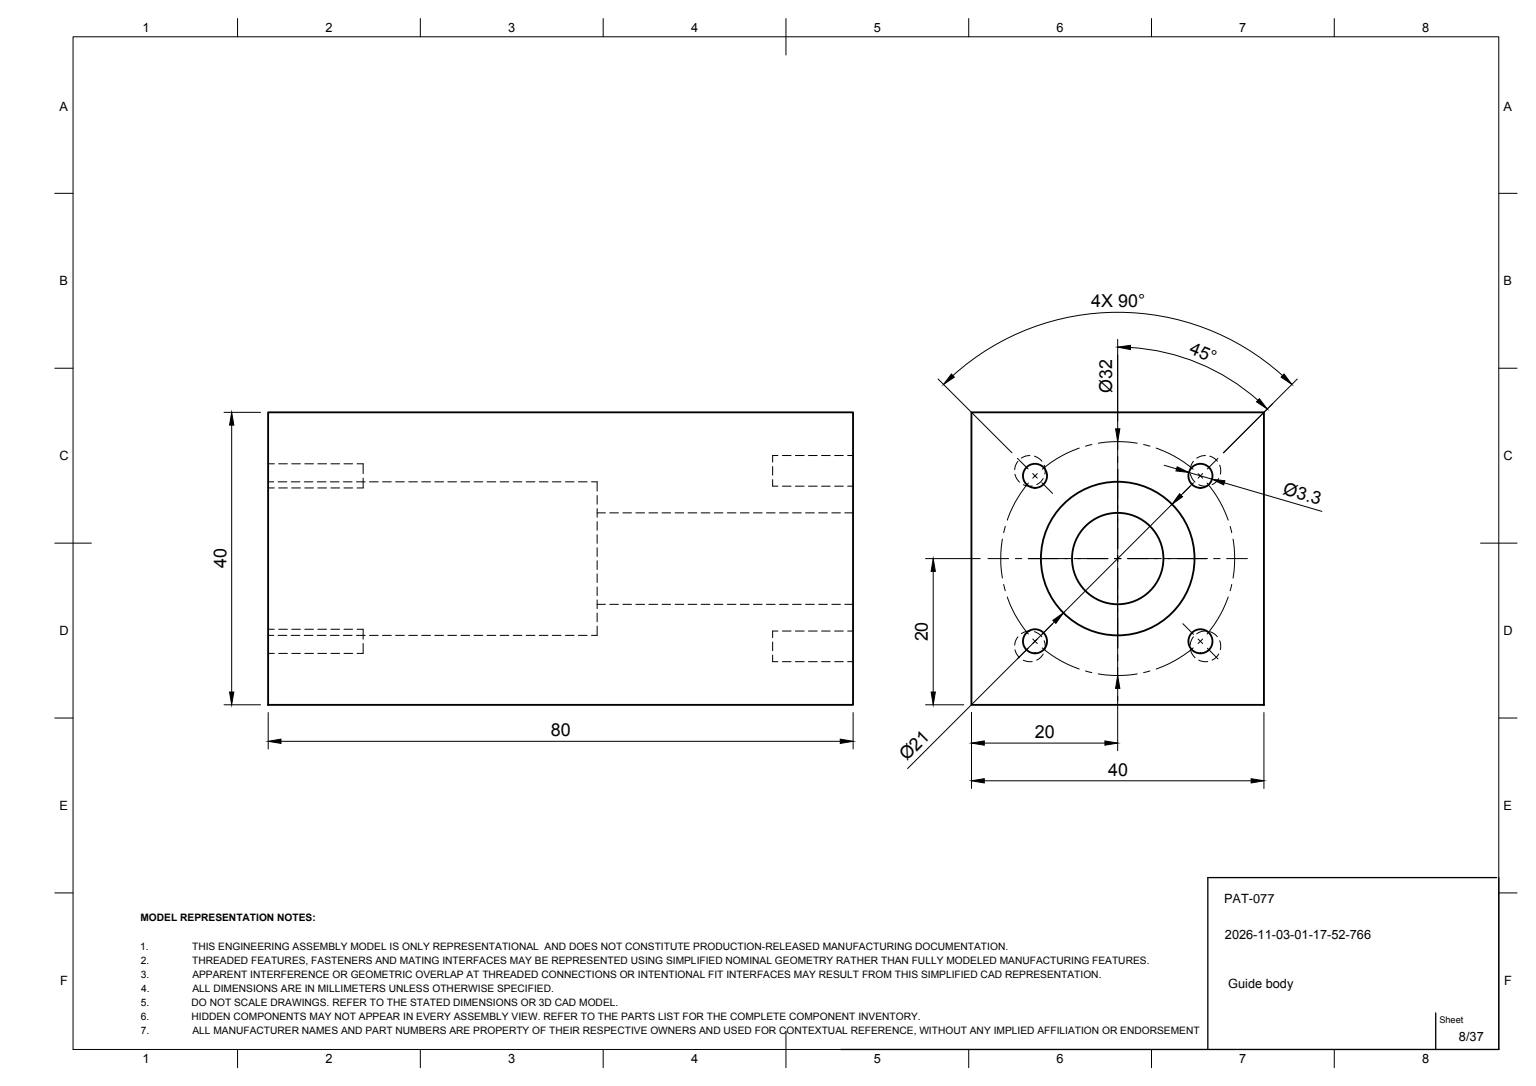
ISO-10303-21;
HEADER;
/* Generated by software containing ST-Developer
 * from STEP Tools, Inc. (www.steptools.com) 
 */

FILE_DESCRIPTION(
/* description */ ('Pallet stop with pneumatic fitting'),
/* implementation_level */ '2;1');

FILE_NAME(
/* name */ 'Guide body.step',
/* time_stamp */ '2026-10-27T10:51:41-07:00',
/* author */ (''),
/* organization */ (''),
/* preprocessor_version */ 'ST-DEVELOPER v20.2',
/* originating_system */ 'Autodesk Translation Framework v15.17.0.0',
/* authorisation */ '');

FILE_SCHEMA (('AUTOMOTIVE_DESIGN { 1 0 10303 214 3 1 1 }'));
ENDSEC;

DATA;
#10=MECHANICAL_DESIGN_GEOMETRIC_PRESENTATION_REPRESENTATION('',(#360),#10265);
#296=SHAPE_REPRESENTATION_RELATIONSHIP('SRR','None',#10409,#328);
#328=ADVANCED_BREP_SHAPE_REPRESENTATION('',(#392),#10233);
#360=STYLED_ITEM('',(#10634),#392);
#392=MANIFOLD_SOLID_BREP('Body1',#5048);
#437=FACE_BOUND('',#1113,.T.);
#438=FACE_BOUND('',#1120,.T.);
#439=FACE_BOUND('',#1121,.T.);
#440=FACE_BOUND('',#1122,.T.);
#441=FACE_BOUND('',#1123,.T.);
#442=FACE_BOUND('',#1124,.T.);
#443=FACE_BOUND('',#1126,.T.);
#444=FACE_BOUND('',#1127,.T.);
#445=FACE_BOUND('',#1128,.T.);
#446=FACE_BOUND('',#1129,.T.);
#447=FACE_BOUND('',#1130,.T.);
#563=PLANE('',#5486);
#564=PLANE('',#5490);
#565=PLANE('',#5494);
#566=PLANE('',#5498);
#567=PLANE('',#5502);
#568=PLANE('',#5506);
#569=PLANE('',#5510);
#570=PLANE('',#5514);
#571=PLANE('',#5518);
#572=PLANE('',#5522);
#573=PLANE('',#5523);
#574=PLANE('',#5524);
#575=PLANE('',#5525);
#576=PLANE('',#5526);
#577=PLANE('',#5527);
#763=FACE_OUTER_BOUND('',#1095,.T.);
#764=FACE_OUTER_BOUND('',#1096,.T.);
#765=FACE_OUTER_BOUND('',#1097,.T.);
#766=FACE_OUTER_BOUND('',#1098,.T.);
#767=FACE_OUTER_BOUND('',#1099,.T.);
#768=FACE_OUTER_BOUND('',#1100,.T.);
#769=FACE_OUTER_BOUND('',#1101,.T.);
#770=FACE_OUTER_BOUND('',#1102,.T.);
#771=FACE_OUTER_BOUND('',#1103,.T.);
#772=FACE_OUTER_BOUND('',#1104,.T.);
#773=FACE_OUTER_BOUND('',#1105,.T.);
#774=FACE_OUTER_BOUND('',#1106,.T.);
#775=FACE_OUTER_BOUND('',#1107,.T.);
#776=FACE_OUTER_BOUND('',#1108,.T.);
#777=FACE_OUTER_BOUND('',#1109,.T.);
#778=FACE_OUTER_BOUND('',#1110,.T.);
#779=FACE_OUTER_BOUND('',#1111,.T.);
#780=FACE_OUTER_BOUND('',#1112,.T.);
#781=FACE_OUTER_BOUND('',#1114,.T.);
#782=FACE_OUTER_BOUND('',#1115,.T.);
#783=FACE_OUTER_BOUND('',#1116,.T.);
#784=FACE_OUTER_BOUND('',#1117,.T.);
#785=FACE_OUTER_BOUND('',#1118,.T.);
#786=FACE_OUTER_BOUND('',#1119,.T.);
#787=FACE_OUTER_BOUND('',#1125,.T.);
#1095=EDGE_LOOP('',(#3536,#3537,#3538,#3539));
#1096=EDGE_LOOP('',(#3540));
#1097=EDGE_LOOP('',(#3541,#3542,#3543,#3544));
#1098=EDGE_LOOP('',(#3545));
#1099=EDGE_LOOP('',(#3546,#3547,#3548,#3549));
#1100=EDGE_LOOP('',(#3550));
#1101=EDGE_LOOP('',(#3551,#3552,#3553,#3554));
#1102=EDGE_LOOP('',(#3555));
#1103=EDGE_LOOP('',(#3556,#3557,#3558,#3559));
#1104=EDGE_LOOP('',(#3560));
#1105=EDGE_LOOP('',(#3561,#3562,#3563,#3564));
#1106=EDGE_LOOP('',(#3565));
#1107=EDGE_LOOP('',(#3566,#3567,#3568,#3569));
#1108=EDGE_LOOP('',(#3570));
#1109=EDGE_LOOP('',(#3571,#3572,#3573,#3574));
#1110=EDGE_LOOP('',(#3575));
#1111=EDGE_LOOP('',(#3576,#3577,#3578,#3579));
#1112=EDGE_LOOP('',(#3580));
#1113=EDGE_LOOP('',(#3581));
#1114=EDGE_LOOP('',(#3582,#3583,#3584,#3585));
#1115=EDGE_LOOP('',(#3586,#3587,#3588,#3589));
#1116=EDGE_LOOP('',(#3590,#3591,#3592,#3593));
#1117=EDGE_LOOP('',(#3594,#3595,#3596,#3597));
#1118=EDGE_LOOP('',(#3598,#3599,#3600,#3601));
#1119=EDGE_LOOP('',(#3602,#3603,#3604,#3605));
#1120=EDGE_LOOP('',(#3606));
#1121=EDGE_LOOP('',(#3607));
#1122=EDGE_LOOP('',(#3608));
#1123=EDGE_LOOP('',(#3609));
#1124=EDGE_LOOP('',(#3610));
#1125=EDGE_LOOP('',(#3611,#3612,#3613,#3614));
#1126=EDGE_LOOP('',(#3615));
#1127=EDGE_LOOP('',(#3616));
#1128=EDGE_LOOP('',(#3617));
#1129=EDGE_LOOP('',(#3618));
#1130=EDGE_LOOP('',(#3619));
#1535=LINE('',#7880,#1870);
#1536=LINE('',#7887,#1871);
#1537=LINE('',#7894,#1872);
#1538=LINE('',#7901,#1873);
#1539=LINE('',#7908,#1874);
#1540=LINE('',#7915,#1875);
#1541=LINE('',#7922,#1876);
#1542=LINE('',#7929,#1877);
#1543=LINE('',#7936,#1878);
#1544=LINE('',#7944,#1879);
#1545=LINE('',#7948,#1880);
#1546=LINE('',#7950,#1881);
#1547=LINE('',#7952,#1882);
#1548=LINE('',#7953,#1883);
#1549=LINE('',#7956,#1884);
#1550=LINE('',#7958,#1885);
#1551=LINE('',#7959,#1886);
#1552=LINE('',#7962,#1887);
#1553=LINE('',#7964,#1888);
#1554=LINE('',#7965,#1889);
#1555=LINE('',#7967,#1890);
#1556=LINE('',#7968,#1891);
#1870=VECTOR('',#6240,0.165);
#1871=VECTOR('',#6249,0.165);
#1872=VECTOR('',#6258,0.165);
#1873=VECTOR('',#6267,0.165);
#1874=VECTOR('',#6276,0.21);
#1875=VECTOR('',#6285,0.21);
#1876=VECTOR('',#6294,0.21);
#1877=VECTOR('',#6303,0.21);
#1878=VECTOR('',#6312,1.05);
#1879=VECTOR('',#6323,0.625);
#1880=VECTOR('',#6326,1.);
#1881=VECTOR('',#6327,1.);
#1882=VECTOR('',#6328,1.);
#1883=VECTOR('',#6329,1.);
#1884=VECTOR('',#6332,1.);
#1885=VECTOR('',#6333,1.);
#1886=VECTOR('',#6334,1.);
#1887=VECTOR('',#6337,1.);
#1888=VECTOR('',#6338,1.);
#1889=VECTOR('',#6339,1.);
#1890=VECTOR('',#6342,1.);
#1891=VECTOR('',#6343,1.);
#2178=CIRCLE('',#5484,0.165);
#2179=CIRCLE('',#5485,0.165);
#2180=CIRCLE('',#5488,0.165);
#2181=CIRCLE('',#5489,0.165);
#2182=CIRCLE('',#5492,0.165);
#2183=CIRCLE('',#5493,0.165);
#2184=CIRCLE('',#5496,0.165);
#2185=CIRCLE('',#5497,0.165);
#2186=CIRCLE('',#5500,0.21);
#2187=CIRCLE('',#5501,0.21);
#2188=CIRCLE('',#5504,0.21);
#2189=CIRCLE('',#5505,0.21);
#2190=CIRCLE('',#5508,0.21);
#2191=CIRCLE('',#5509,0.21);
#2192=CIRCLE('',#5512,0.21);
#2193=CIRCLE('',#5513,0.21);
#2194=CIRCLE('',#5516,1.05);
#2195=CIRCLE('',#5517,1.05);
#2196=CIRCLE('',#5519,0.625);
#2197=CIRCLE('',#5521,0.625);
#2449=VERTEX_POINT('',#7877);
#2450=VERTEX_POINT('',#7879);
#2451=VERTEX_POINT('',#7884);
#2452=VERTEX_POINT('',#7886);
#2453=VERTEX_POINT('',#7891);
#2454=VERTEX_POINT('',#7893);
#2455=VERTEX_POINT('',#7898);
#2456=VERTEX_POINT('',#7900);
#2457=VERTEX_POINT('',#7905);
#2458=VERTEX_POINT('',#7907);
#2459=VERTEX_POINT('',#7912);
#2460=VERTEX_POINT('',#7914);
#2461=VERTEX_POINT('',#7919);
#2462=VERTEX_POINT('',#7921);
#2463=VERTEX_POINT('',#7926);
#2464=VERTEX_POINT('',#7928);
#2465=VERTEX_POINT('',#7933);
#2466=VERTEX_POINT('',#7935);
#2467=VERTEX_POINT('',#7939);
#2468=VERTEX_POINT('',#7942);
#2469=VERTEX_POINT('',#7946);
#2470=VERTEX_POINT('',#7947);
#2471=VERTEX_POINT('',#7949);
#2472=VERTEX_POINT('',#7951);
#2473=VERTEX_POINT('',#7955);
#2474=VERTEX_POINT('',#7957);
#2475=VERTEX_POINT('',#7961);
#2476=VERTEX_POINT('',#7963);
#2867=EDGE_CURVE('',#2449,#2449,#2178,.T.);
#2868=EDGE_CURVE('',#2449,#2450,#1535,.T.);
#2869=EDGE_CURVE('',#2450,#2450,#2179,.T.);
#2870=EDGE_CURVE('',#2451,#2451,#2180,.T.);
#2871=EDGE_CURVE('',#2451,#2452,#1536,.T.);
#2872=EDGE_CURVE('',#2452,#2452,#2181,.T.);
#2873=EDGE_CURVE('',#2453,#2453,#2182,.T.);
#2874=EDGE_CURVE('',#2453,#2454,#1537,.T.);
#2875=EDGE_CURVE('',#2454,#2454,#2183,.T.);
#2876=EDGE_CURVE('',#2455,#2455,#2184,.T.);
#2877=EDGE_CURVE('',#2455,#2456,#1538,.T.);
#2878=EDGE_CURVE('',#2456,#2456,#2185,.T.);
#2879=EDGE_CURVE('',#2457,#2457,#2186,.T.);
#2880=EDGE_CURVE('',#2457,#2458,#1539,.T.);
#2881=EDGE_CURVE('',#2458,#2458,#2187,.T.);
#2882=EDGE_CURVE('',#2459,#2459,#2188,.T.);
#2883=EDGE_CURVE('',#2459,#2460,#1540,.T.);
#2884=EDGE_CURVE('',#2460,#2460,#2189,.T.);
#2885=EDGE_CURVE('',#2461,#2461,#2190,.T.);
#2886=EDGE_CURVE('',#2461,#2462,#1541,.T.);
#2887=EDGE_CURVE('',#2462,#2462,#2191,.T.);
#2888=EDGE_CURVE('',#2463,#2463,#2192,.T.);
#2889=EDGE_CURVE('',#2463,#2464,#1542,.T.);
#2890=EDGE_CURVE('',#2464,#2464,#2193,.T.);
#2891=EDGE_CURVE('',#2465,#2465,#2194,.T.);
#2892=EDGE_CURVE('',#2465,#2466,#1543,.T.);
#2893=EDGE_CURVE('',#2466,#2466,#2195,.T.);
#2894=EDGE_CURVE('',#2467,#2467,#2196,.T.);
#2895=EDGE_CURVE('',#2468,#2468,#2197,.T.);
#2896=EDGE_CURVE('',#2468,#2467,#1544,.T.);
#2897=EDGE_CURVE('',#2469,#2470,#1545,.T.);
#2898=EDGE_CURVE('',#2470,#2471,#1546,.T.);
#2899=EDGE_CURVE('',#2472,#2471,#1547,.T.);
#2900=EDGE_CURVE('',#2469,#2472,#1548,.T.);
#2901=EDGE_CURVE('',#2473,#2469,#1549,.T.);
#2902=EDGE_CURVE('',#2474,#2472,#1550,.T.);
#2903=EDGE_CURVE('',#2473,#2474,#1551,.T.);
#2904=EDGE_CURVE('',#2475,#2473,#1552,.T.);
#2905=EDGE_CURVE('',#2476,#2474,#1553,.T.);
#2906=EDGE_CURVE('',#2475,#2476,#1554,.T.);
#2907=EDGE_CURVE('',#2470,#2475,#1555,.T.);
#2908=EDGE_CURVE('',#2471,#2476,#1556,.T.);
#3536=ORIENTED_EDGE('',*,*,#2867,.F.);
#3537=ORIENTED_EDGE('',*,*,#2868,.T.);
#3538=ORIENTED_EDGE('',*,*,#2869,.F.);
#3539=ORIENTED_EDGE('',*,*,#2868,.F.);
#3540=ORIENTED_EDGE('',*,*,#2867,.T.);
#3541=ORIENTED_EDGE('',*,*,#2870,.F.);
#3542=ORIENTED_EDGE('',*,*,#2871,.T.);
#3543=ORIENTED_EDGE('',*,*,#2872,.F.);
#3544=ORIENTED_EDGE('',*,*,#2871,.F.);
#3545=ORIENTED_EDGE('',*,*,#2870,.T.);
#3546=ORIENTED_EDGE('',*,*,#2873,.F.);
#3547=ORIENTED_EDGE('',*,*,#2874,.T.);
#3548=ORIENTED_EDGE('',*,*,#2875,.F.);
#3549=ORIENTED_EDGE('',*,*,#2874,.F.);
#3550=ORIENTED_EDGE('',*,*,#2873,.T.);
#3551=ORIENTED_EDGE('',*,*,#2876,.F.);
#3552=ORIENTED_EDGE('',*,*,#2877,.T.);
#3553=ORIENTED_EDGE('',*,*,#2878,.F.);
#3554=ORIENTED_EDGE('',*,*,#2877,.F.);
#3555=ORIENTED_EDGE('',*,*,#2876,.T.);
#3556=ORIENTED_EDGE('',*,*,#2879,.F.);
#3557=ORIENTED_EDGE('',*,*,#2880,.T.);
#3558=ORIENTED_EDGE('',*,*,#2881,.T.);
#3559=ORIENTED_EDGE('',*,*,#2880,.F.);
#3560=ORIENTED_EDGE('',*,*,#2881,.F.);
#3561=ORIENTED_EDGE('',*,*,#2882,.F.);
#3562=ORIENTED_EDGE('',*,*,#2883,.T.);
#3563=ORIENTED_EDGE('',*,*,#2884,.T.);
#3564=ORIENTED_EDGE('',*,*,#2883,.F.);
#3565=ORIENTED_EDGE('',*,*,#2884,.F.);
#3566=ORIENTED_EDGE('',*,*,#2885,.F.);
#3567=ORIENTED_EDGE('',*,*,#2886,.T.);
#3568=ORIENTED_EDGE('',*,*,#2887,.T.);
#3569=ORIENTED_EDGE('',*,*,#2886,.F.);
#3570=ORIENTED_EDGE('',*,*,#2887,.F.);
#3571=ORIENTED_EDGE('',*,*,#2888,.F.);
#3572=ORIENTED_EDGE('',*,*,#2889,.T.);
#3573=ORIENTED_EDGE('',*,*,#2890,.T.);
#3574=ORIENTED_EDGE('',*,*,#2889,.F.);
#3575=ORIENTED_EDGE('',*,*,#2890,.F.);
#3576=ORIENTED_EDGE('',*,*,#2891,.F.);
#3577=ORIENTED_EDGE('',*,*,#2892,.T.);
#3578=ORIENTED_EDGE('',*,*,#2893,.F.);
#3579=ORIENTED_EDGE('',*,*,#2892,.F.);
#3580=ORIENTED_EDGE('',*,*,#2891,.T.);
#3581=ORIENTED_EDGE('',*,*,#2894,.F.);
#3582=ORIENTED_EDGE('',*,*,#2895,.F.);
#3583=ORIENTED_EDGE('',*,*,#2896,.T.);
#3584=ORIENTED_EDGE('',*,*,#2894,.T.);
#3585=ORIENTED_EDGE('',*,*,#2896,.F.);
#3586=ORIENTED_EDGE('',*,*,#2897,.T.);
#3587=ORIENTED_EDGE('',*,*,#2898,.T.);
#3588=ORIENTED_EDGE('',*,*,#2899,.F.);
#3589=ORIENTED_EDGE('',*,*,#2900,.F.);
#3590=ORIENTED_EDGE('',*,*,#2901,.T.);
#3591=ORIENTED_EDGE('',*,*,#2900,.T.);
#3592=ORIENTED_EDGE('',*,*,#2902,.F.);
#3593=ORIENTED_EDGE('',*,*,#2903,.F.);
#3594=ORIENTED_EDGE('',*,*,#2904,.T.);
#3595=ORIENTED_EDGE('',*,*,#2903,.T.);
#3596=ORIENTED_EDGE('',*,*,#2905,.F.);
#3597=ORIENTED_EDGE('',*,*,#2906,.F.);
#3598=ORIENTED_EDGE('',*,*,#2907,.T.);
#3599=ORIENTED_EDGE('',*,*,#2906,.T.);
#3600=ORIENTED_EDGE('',*,*,#2908,.F.);
#3601=ORIENTED_EDGE('',*,*,#2898,.F.);
#3602=ORIENTED_EDGE('',*,*,#2908,.T.);
#3603=ORIENTED_EDGE('',*,*,#2905,.T.);
#3604=ORIENTED_EDGE('',*,*,#2902,.T.);
#3605=ORIENTED_EDGE('',*,*,#2899,.T.);
#3606=ORIENTED_EDGE('',*,*,#2893,.T.);
#3607=ORIENTED_EDGE('',*,*,#2878,.T.);
#3608=ORIENTED_EDGE('',*,*,#2875,.T.);
#3609=ORIENTED_EDGE('',*,*,#2872,.T.);
#3610=ORIENTED_EDGE('',*,*,#2869,.T.);
#3611=ORIENTED_EDGE('',*,*,#2907,.F.);
#3612=ORIENTED_EDGE('',*,*,#2897,.F.);
#3613=ORIENTED_EDGE('',*,*,#2901,.F.);
#3614=ORIENTED_EDGE('',*,*,#2904,.F.);
#3615=ORIENTED_EDGE('',*,*,#2895,.T.);
#3616=ORIENTED_EDGE('',*,*,#2888,.T.);
#3617=ORIENTED_EDGE('',*,*,#2885,.T.);
#3618=ORIENTED_EDGE('',*,*,#2882,.T.);
#3619=ORIENTED_EDGE('',*,*,#2879,.T.);
#4631=CYLINDRICAL_SURFACE('',#5483,0.165);
#4632=CYLINDRICAL_SURFACE('',#5487,0.165);
#4633=CYLINDRICAL_SURFACE('',#5491,0.165);
#4634=CYLINDRICAL_SURFACE('',#5495,0.165);
#4635=CYLINDRICAL_SURFACE('',#5499,0.21);
#4636=CYLINDRICAL_SURFACE('',#5503,0.21);
#4637=CYLINDRICAL_SURFACE('',#5507,0.21);
#4638=CYLINDRICAL_SURFACE('',#5511,0.21);
#4639=CYLINDRICAL_SURFACE('',#5515,1.05);
#4640=CYLINDRICAL_SURFACE('',#5520,0.625);
#4758=ADVANCED_FACE('',(#763),#4631,.F.);
#4759=ADVANCED_FACE('',(#764),#563,.T.);
#4760=ADVANCED_FACE('',(#765),#4632,.F.);
#4761=ADVANCED_FACE('',(#766),#564,.T.);
#4762=ADVANCED_FACE('',(#767),#4633,.F.);
#4763=ADVANCED_FACE('',(#768),#565,.T.);
#4764=ADVANCED_FACE('',(#769),#4634,.F.);
#4765=ADVANCED_FACE('',(#770),#566,.T.);
#4766=ADVANCED_FACE('',(#771),#4635,.F.);
#4767=ADVANCED_FACE('',(#772),#567,.F.);
#4768=ADVANCED_FACE('',(#773),#4636,.F.);
#4769=ADVANCED_FACE('',(#774),#568,.F.);
#4770=ADVANCED_FACE('',(#775),#4637,.F.);
#4771=ADVANCED_FACE('',(#776),#569,.F.);
#4772=ADVANCED_FACE('',(#777),#4638,.F.);
#4773=ADVANCED_FACE('',(#778),#570,.F.);
#4774=ADVANCED_FACE('',(#779),#4639,.F.);
#4775=ADVANCED_FACE('',(#780,#437),#571,.T.);
#4776=ADVANCED_FACE('',(#781),#4640,.F.);
#4777=ADVANCED_FACE('',(#782),#572,.T.);
#4778=ADVANCED_FACE('',(#783),#573,.T.);
#4779=ADVANCED_FACE('',(#784),#574,.T.);
#4780=ADVANCED_FACE('',(#785),#575,.T.);
#4781=ADVANCED_FACE('',(#786,#438,#439,#440,#441,#442),#576,.T.);
#4782=ADVANCED_FACE('',(#787,#443,#444,#445,#446,#447),#577,.F.);
#5048=CLOSED_SHELL('',(#4758,#4759,#4760,#4761,#4762,#4763,#4764,#4765,
#4766,#4767,#4768,#4769,#4770,#4771,#4772,#4773,#4774,#4775,#4776,#4777,
#4778,#4779,#4780,#4781,#4782));
#5482=AXIS2_PLACEMENT_3D('',#7875,#6234,#6235);
#5483=AXIS2_PLACEMENT_3D('',#7876,#6236,#6237);
#5484=AXIS2_PLACEMENT_3D('',#7878,#6238,#6239);
#5485=AXIS2_PLACEMENT_3D('',#7881,#6241,#6242);
#5486=AXIS2_PLACEMENT_3D('',#7882,#6243,#6244);
#5487=AXIS2_PLACEMENT_3D('',#7883,#6245,#6246);
#5488=AXIS2_PLACEMENT_3D('',#7885,#6247,#6248);
#5489=AXIS2_PLACEMENT_3D('',#7888,#6250,#6251);
#5490=AXIS2_PLACEMENT_3D('',#7889,#6252,#6253);
#5491=AXIS2_PLACEMENT_3D('',#7890,#6254,#6255);
#5492=AXIS2_PLACEMENT_3D('',#7892,#6256,#6257);
#5493=AXIS2_PLACEMENT_3D('',#7895,#6259,#6260);
#5494=AXIS2_PLACEMENT_3D('',#7896,#6261,#6262);
#5495=AXIS2_PLACEMENT_3D('',#7897,#6263,#6264);
#5496=AXIS2_PLACEMENT_3D('',#7899,#6265,#6266);
#5497=AXIS2_PLACEMENT_3D('',#7902,#6268,#6269);
#5498=AXIS2_PLACEMENT_3D('',#7903,#6270,#6271);
#5499=AXIS2_PLACEMENT_3D('',#7904,#6272,#6273);
#5500=AXIS2_PLACEMENT_3D('',#7906,#6274,#6275);
#5501=AXIS2_PLACEMENT_3D('',#7909,#6277,#6278);
#5502=AXIS2_PLACEMENT_3D('',#7910,#6279,#6280);
#5503=AXIS2_PLACEMENT_3D('',#7911,#6281,#6282);
#5504=AXIS2_PLACEMENT_3D('',#7913,#6283,#6284);
#5505=AXIS2_PLACEMENT_3D('',#7916,#6286,#6287);
#5506=AXIS2_PLACEMENT_3D('',#7917,#6288,#6289);
#5507=AXIS2_PLACEMENT_3D('',#7918,#6290,#6291);
#5508=AXIS2_PLACEMENT_3D('',#7920,#6292,#6293);
#5509=AXIS2_PLACEMENT_3D('',#7923,#6295,#6296);
#5510=AXIS2_PLACEMENT_3D('',#7924,#6297,#6298);
#5511=AXIS2_PLACEMENT_3D('',#7925,#6299,#6300);
#5512=AXIS2_PLACEMENT_3D('',#7927,#6301,#6302);
#5513=AXIS2_PLACEMENT_3D('',#7930,#6304,#6305);
#5514=AXIS2_PLACEMENT_3D('',#7931,#6306,#6307);
#5515=AXIS2_PLACEMENT_3D('',#7932,#6308,#6309);
#5516=AXIS2_PLACEMENT_3D('',#7934,#6310,#6311);
#5517=AXIS2_PLACEMENT_3D('',#7937,#6313,#6314);
#5518=AXIS2_PLACEMENT_3D('',#7938,#6315,#6316);
#5519=AXIS2_PLACEMENT_3D('',#7940,#6317,#6318);
#5520=AXIS2_PLACEMENT_3D('',#7941,#6319,#6320);
#5521=AXIS2_PLACEMENT_3D('',#7943,#6321,#6322);
#5522=AXIS2_PLACEMENT_3D('',#7945,#6324,#6325);
#5523=AXIS2_PLACEMENT_3D('',#7954,#6330,#6331);
#5524=AXIS2_PLACEMENT_3D('',#7960,#6335,#6336);
#5525=AXIS2_PLACEMENT_3D('',#7966,#6340,#6341);
#5526=AXIS2_PLACEMENT_3D('',#7969,#6344,#6345);
#5527=AXIS2_PLACEMENT_3D('',#7970,#6346,#6347);
#6234=DIRECTION('axis',(0.,0.,1.));
#6235=DIRECTION('refdir',(1.,0.,0.));
#6236=DIRECTION('center_axis',(0.,0.,1.));
#6237=DIRECTION('ref_axis',(1.,0.,0.));
#6238=DIRECTION('center_axis',(0.,0.,1.));
#6239=DIRECTION('ref_axis',(1.,0.,0.));
#6240=DIRECTION('',(0.,0.,1.));
#6241=DIRECTION('center_axis',(0.,0.,-1.));
#6242=DIRECTION('ref_axis',(1.,0.,0.));
#6243=DIRECTION('center_axis',(0.,0.,1.));
#6244=DIRECTION('ref_axis',(1.,0.,0.));
#6245=DIRECTION('center_axis',(0.,0.,1.));
#6246=DIRECTION('ref_axis',(1.,0.,0.));
#6247=DIRECTION('center_axis',(0.,0.,1.));
#6248=DIRECTION('ref_axis',(1.,0.,0.));
#6249=DIRECTION('',(0.,0.,1.));
#6250=DIRECTION('center_axis',(0.,0.,-1.));
#6251=DIRECTION('ref_axis',(1.,0.,0.));
#6252=DIRECTION('center_axis',(0.,0.,1.));
#6253=DIRECTION('ref_axis',(1.,0.,0.));
#6254=DIRECTION('center_axis',(0.,0.,1.));
#6255=DIRECTION('ref_axis',(1.,0.,0.));
#6256=DIRECTION('center_axis',(0.,0.,1.));
#6257=DIRECTION('ref_axis',(1.,0.,0.));
#6258=DIRECTION('',(0.,0.,1.));
#6259=DIRECTION('center_axis',(0.,0.,-1.));
#6260=DIRECTION('ref_axis',(1.,0.,0.));
#6261=DIRECTION('center_axis',(0.,0.,1.));
#6262=DIRECTION('ref_axis',(1.,0.,0.));
#6263=DIRECTION('center_axis',(0.,0.,1.));
#6264=DIRECTION('ref_axis',(1.,0.,0.));
#6265=DIRECTION('center_axis',(0.,0.,1.));
#6266=DIRECTION('ref_axis',(1.,0.,0.));
#6267=DIRECTION('',(0.,0.,1.));
#6268=DIRECTION('center_axis',(0.,0.,-1.));
#6269=DIRECTION('ref_axis',(1.,0.,0.));
#6270=DIRECTION('center_axis',(0.,0.,1.));
#6271=DIRECTION('ref_axis',(1.,0.,0.));
#6272=DIRECTION('center_axis',(0.,0.,1.));
#6273=DIRECTION('ref_axis',(1.,0.,0.));
#6274=DIRECTION('center_axis',(0.,0.,1.));
#6275=DIRECTION('ref_axis',(1.,0.,0.));
#6276=DIRECTION('',(0.,0.,1.));
#6277=DIRECTION('center_axis',(0.,0.,1.));
#6278=DIRECTION('ref_axis',(1.,0.,0.));
#6279=DIRECTION('center_axis',(0.,0.,1.));
#6280=DIRECTION('ref_axis',(1.,0.,0.));
#6281=DIRECTION('center_axis',(0.,0.,1.));
#6282=DIRECTION('ref_axis',(1.,0.,0.));
#6283=DIRECTION('center_axis',(0.,0.,1.));
#6284=DIRECTION('ref_axis',(1.,0.,0.));
#6285=DIRECTION('',(0.,0.,1.));
#6286=DIRECTION('center_axis',(0.,0.,1.));
#6287=DIRECTION('ref_axis',(1.,0.,0.));
#6288=DIRECTION('center_axis',(0.,0.,1.));
#6289=DIRECTION('ref_axis',(1.,0.,0.));
#6290=DIRECTION('center_axis',(0.,0.,1.));
#6291=DIRECTION('ref_axis',(1.,0.,0.));
#6292=DIRECTION('center_axis',(0.,0.,1.));
#6293=DIRECTION('ref_axis',(1.,0.,0.));
#6294=DIRECTION('',(0.,0.,1.));
#6295=DIRECTION('center_axis',(0.,0.,1.));
#6296=DIRECTION('ref_axis',(1.,0.,0.));
#6297=DIRECTION('center_axis',(0.,0.,1.));
#6298=DIRECTION('ref_axis',(1.,0.,0.));
#6299=DIRECTION('center_axis',(0.,0.,1.));
#6300=DIRECTION('ref_axis',(1.,0.,0.));
#6301=DIRECTION('center_axis',(0.,0.,1.));
#6302=DIRECTION('ref_axis',(1.,0.,0.));
#6303=DIRECTION('',(0.,0.,1.));
#6304=DIRECTION('center_axis',(0.,0.,1.));
#6305=DIRECTION('ref_axis',(1.,0.,0.));
#6306=DIRECTION('center_axis',(0.,0.,1.));
#6307=DIRECTION('ref_axis',(1.,0.,0.));
#6308=DIRECTION('center_axis',(0.,0.,1.));
#6309=DIRECTION('ref_axis',(1.,0.,0.));
#6310=DIRECTION('center_axis',(0.,0.,1.));
#6311=DIRECTION('ref_axis',(1.,0.,0.));
#6312=DIRECTION('',(0.,0.,1.));
#6313=DIRECTION('center_axis',(0.,0.,-1.));
#6314=DIRECTION('ref_axis',(1.,0.,0.));
#6315=DIRECTION('center_axis',(0.,0.,1.));
#6316=DIRECTION('ref_axis',(1.,0.,0.));
#6317=DIRECTION('center_axis',(0.,0.,1.));
#6318=DIRECTION('ref_axis',(1.,0.,0.));
#6319=DIRECTION('center_axis',(0.,0.,1.));
#6320=DIRECTION('ref_axis',(1.,0.,0.));
#6321=DIRECTION('center_axis',(0.,0.,1.));
#6322=DIRECTION('ref_axis',(1.,0.,0.));
#6323=DIRECTION('',(0.,0.,1.));
#6324=DIRECTION('center_axis',(0.,1.,0.));
#6325=DIRECTION('ref_axis',(-1.,0.,0.));
#6326=DIRECTION('',(-1.,0.,0.));
#6327=DIRECTION('',(0.,0.,1.));
#6328=DIRECTION('',(-1.,0.,0.));
#6329=DIRECTION('',(0.,0.,1.));
#6330=DIRECTION('center_axis',(1.,0.,0.));
#6331=DIRECTION('ref_axis',(0.,1.,0.));
#6332=DIRECTION('',(0.,1.,0.));
#6333=DIRECTION('',(0.,1.,0.));
#6334=DIRECTION('',(0.,0.,1.));
#6335=DIRECTION('center_axis',(0.,-1.,0.));
#6336=DIRECTION('ref_axis',(1.,0.,0.));
#6337=DIRECTION('',(1.,0.,0.));
#6338=DIRECTION('',(1.,0.,0.));
#6339=DIRECTION('',(0.,0.,1.));
#6340=DIRECTION('center_axis',(-1.,0.,0.));
#6341=DIRECTION('ref_axis',(0.,-1.,0.));
#6342=DIRECTION('',(0.,-1.,0.));
#6343=DIRECTION('',(0.,-1.,0.));
#6344=DIRECTION('center_axis',(0.,0.,1.));
#6345=DIRECTION('ref_axis',(1.,0.,0.));
#6346=DIRECTION('center_axis',(0.,0.,1.));
#6347=DIRECTION('ref_axis',(1.,0.,0.));
#7875=CARTESIAN_POINT('',(0.,0.,0.));
#7876=CARTESIAN_POINT('Origin',(-1.13137084989848,-1.13137084989848,6.7));
#7877=CARTESIAN_POINT('',(-1.29637084989848,-1.13137084989848,6.7));
#7878=CARTESIAN_POINT('Origin',(-1.13137084989848,-1.13137084989848,6.7));
#7879=CARTESIAN_POINT('',(-1.29637084989848,-1.13137084989848,8.));
#7880=CARTESIAN_POINT('',(-1.29637084989848,-1.13137084989848,6.7));
#7881=CARTESIAN_POINT('Origin',(-1.13137084989848,-1.13137084989848,8.));
#7882=CARTESIAN_POINT('Origin',(-1.13137084989848,-1.13137084989848,6.7));
#7883=CARTESIAN_POINT('Origin',(-1.13137084989848,1.13137084989848,6.7));
#7884=CARTESIAN_POINT('',(-1.29637084989848,1.13137084989848,6.7));
#7885=CARTESIAN_POINT('Origin',(-1.13137084989848,1.13137084989848,6.7));
#7886=CARTESIAN_POINT('',(-1.29637084989848,1.13137084989848,8.));
#7887=CARTESIAN_POINT('',(-1.29637084989848,1.13137084989848,6.7));
#7888=CARTESIAN_POINT('Origin',(-1.13137084989848,1.13137084989848,8.));
#7889=CARTESIAN_POINT('Origin',(-1.13137084989848,1.13137084989848,6.7));
#7890=CARTESIAN_POINT('Origin',(1.13137084989848,1.13137084989848,6.7));
#7891=CARTESIAN_POINT('',(0.966370849898476,1.13137084989848,6.7));
#7892=CARTESIAN_POINT('Origin',(1.13137084989848,1.13137084989848,6.7));
#7893=CARTESIAN_POINT('',(0.966370849898476,1.13137084989848,8.));
#7894=CARTESIAN_POINT('',(0.966370849898476,1.13137084989848,6.7));
#7895=CARTESIAN_POINT('Origin',(1.13137084989848,1.13137084989848,8.));
#7896=CARTESIAN_POINT('Origin',(1.13137084989848,1.13137084989848,6.7));
#7897=CARTESIAN_POINT('Origin',(1.13137084989848,-1.13137084989848,6.7));
#7898=CARTESIAN_POINT('',(0.966370849898476,-1.13137084989848,6.7));
#7899=CARTESIAN_POINT('Origin',(1.13137084989848,-1.13137084989848,6.7));
#7900=CARTESIAN_POINT('',(0.966370849898476,-1.13137084989848,8.));
#7901=CARTESIAN_POINT('',(0.966370849898476,-1.13137084989848,6.7));
#7902=CARTESIAN_POINT('Origin',(1.13137084989848,-1.13137084989848,8.));
#7903=CARTESIAN_POINT('Origin',(1.13137084989848,-1.13137084989848,6.7));
#7904=CARTESIAN_POINT('Origin',(1.2,-1.2,-0.1));
#7905=CARTESIAN_POINT('',(0.99,-1.2,0.));
#7906=CARTESIAN_POINT('Origin',(1.2,-1.2,0.));
#7907=CARTESIAN_POINT('',(0.99,-1.2,1.1));
#7908=CARTESIAN_POINT('',(0.99,-1.2,-0.1));
#7909=CARTESIAN_POINT('Origin',(1.2,-1.2,1.1));
#7910=CARTESIAN_POINT('Origin',(1.2,-1.2,1.1));
#7911=CARTESIAN_POINT('Origin',(-1.2,1.2,-0.1));
#7912=CARTESIAN_POINT('',(-1.41,1.2,0.));
#7913=CARTESIAN_POINT('Origin',(-1.2,1.2,0.));
#7914=CARTESIAN_POINT('',(-1.41,1.2,1.1));
#7915=CARTESIAN_POINT('',(-1.41,1.2,-0.1));
#7916=CARTESIAN_POINT('Origin',(-1.2,1.2,1.1));
#7917=CARTESIAN_POINT('Origin',(-1.2,1.2,1.1));
#7918=CARTESIAN_POINT('Origin',(-1.2,-1.2,-0.1));
#7919=CARTESIAN_POINT('',(-1.41,-1.2,0.));
#7920=CARTESIAN_POINT('Origin',(-1.2,-1.2,0.));
#7921=CARTESIAN_POINT('',(-1.41,-1.2,1.1));
#7922=CARTESIAN_POINT('',(-1.41,-1.2,-0.1));
#7923=CARTESIAN_POINT('Origin',(-1.2,-1.2,1.1));
#7924=CARTESIAN_POINT('Origin',(-1.2,-1.2,1.1));
#7925=CARTESIAN_POINT('Origin',(1.2,1.2,-0.1));
#7926=CARTESIAN_POINT('',(0.99,1.2,0.));
#7927=CARTESIAN_POINT('Origin',(1.2,1.2,0.));
#7928=CARTESIAN_POINT('',(0.99,1.2,1.1));
#7929=CARTESIAN_POINT('',(0.99,1.2,-0.1));
#7930=CARTESIAN_POINT('Origin',(1.2,1.2,1.1));
#7931=CARTESIAN_POINT('Origin',(1.2,1.2,1.1));
#7932=CARTESIAN_POINT('Origin',(0.,0.,3.5));
#7933=CARTESIAN_POINT('',(-1.05,-1.28587913910472E-16,3.5));
#7934=CARTESIAN_POINT('Origin',(0.,0.,3.5));
#7935=CARTESIAN_POINT('',(-1.05,1.28587913910472E-16,8.));
#7936=CARTESIAN_POINT('',(-1.05,-1.28587913910472E-16,3.5));
#7937=CARTESIAN_POINT('Origin',(0.,0.,8.));
#7938=CARTESIAN_POINT('Origin',(0.,0.,3.5));
#7939=CARTESIAN_POINT('',(-0.625,-7.65404249467096E-17,3.5));
#7940=CARTESIAN_POINT('Origin',(0.,0.,3.5));
#7941=CARTESIAN_POINT('Origin',(0.,0.,-0.1));
#7942=CARTESIAN_POINT('',(-0.625,-7.65404249467096E-17,0.));
#7943=CARTESIAN_POINT('Origin',(0.,0.,0.));
#7944=CARTESIAN_POINT('',(-0.625,-7.65404249467096E-17,-0.1));
#7945=CARTESIAN_POINT('Origin',(2.,2.,0.));
#7946=CARTESIAN_POINT('',(2.,2.,0.));
#7947=CARTESIAN_POINT('',(-2.,2.,0.));
#7948=CARTESIAN_POINT('',(2.,2.,0.));
#7949=CARTESIAN_POINT('',(-2.,2.,8.));
#7950=CARTESIAN_POINT('',(-2.,2.,0.));
#7951=CARTESIAN_POINT('',(2.,2.,8.));
#7952=CARTESIAN_POINT('',(2.,2.,8.));
#7953=CARTESIAN_POINT('',(2.,2.,0.));
#7954=CARTESIAN_POINT('Origin',(2.,-2.,0.));
#7955=CARTESIAN_POINT('',(2.,-2.,0.));
#7956=CARTESIAN_POINT('',(2.,-2.,0.));
#7957=CARTESIAN_POINT('',(2.,-2.,8.));
#7958=CARTESIAN_POINT('',(2.,-2.,8.));
#7959=CARTESIAN_POINT('',(2.,-2.,0.));
#7960=CARTESIAN_POINT('Origin',(-2.,-2.,0.));
#7961=CARTESIAN_POINT('',(-2.,-2.,0.));
#7962=CARTESIAN_POINT('',(-2.,-2.,0.));
#7963=CARTESIAN_POINT('',(-2.,-2.,8.));
#7964=CARTESIAN_POINT('',(-2.,-2.,8.));
#7965=CARTESIAN_POINT('',(-2.,-2.,0.));
#7966=CARTESIAN_POINT('Origin',(-2.,2.,0.));
#7967=CARTESIAN_POINT('',(-2.,2.,0.));
#7968=CARTESIAN_POINT('',(-2.,2.,8.));
#7969=CARTESIAN_POINT('Origin',(0.,0.,8.));
#7970=CARTESIAN_POINT('Origin',(0.,0.,0.));
#10195=UNCERTAINTY_MEASURE_WITH_UNIT(LENGTH_MEASURE(0.001),#10266,
'DISTANCE_ACCURACY_VALUE',
'Maximum model space distance between geometric entities at asserted c
onnectivities');
#10227=UNCERTAINTY_MEASURE_WITH_UNIT(LENGTH_MEASURE(0.001),#10266,
'DISTANCE_ACCURACY_VALUE',
'Maximum model space distance between geometric entities at asserted c
onnectivities');
#10233=(
GEOMETRIC_REPRESENTATION_CONTEXT(3)
GLOBAL_UNCERTAINTY_ASSIGNED_CONTEXT((#10195))
GLOBAL_UNIT_ASSIGNED_CONTEXT((#10266,#10268,#10269))
REPRESENTATION_CONTEXT('','3D')
);
#10265=(
GEOMETRIC_REPRESENTATION_CONTEXT(3)
GLOBAL_UNCERTAINTY_ASSIGNED_CONTEXT((#10227))
GLOBAL_UNIT_ASSIGNED_CONTEXT((#10266,#10268,#10269))
REPRESENTATION_CONTEXT('','3D')
);
#10266=(
LENGTH_UNIT()
NAMED_UNIT(*)
SI_UNIT(.CENTI.,.METRE.)
);
#10268=(
NAMED_UNIT(*)
PLANE_ANGLE_UNIT()
SI_UNIT($,.RADIAN.)
);
#10269=(
NAMED_UNIT(*)
SI_UNIT($,.STERADIAN.)
SOLID_ANGLE_UNIT()
);
#10275=SHAPE_DEFINITION_REPRESENTATION(#10312,#10409);
#10312=PRODUCT_DEFINITION_SHAPE('',$,#10447);
#10409=SHAPE_REPRESENTATION('',(#5482),#10233);
#10441=PRODUCT_DEFINITION_CONTEXT('part definition',#10554,'design');
#10447=PRODUCT_DEFINITION('Guide body','Guide body',#10484,#10441);
#10484=PRODUCT_DEFINITION_FORMATION('',$,#10561);
#10554=APPLICATION_CONTEXT(
'Core Data for Automotive Mechanical Design Process');
#10555=PRODUCT_CONTEXT('part definition',#10554,'mechanical');
#10561=PRODUCT('Guide body','Guide body','Guide body',(#10555));
#10628=COLOUR_RGB('Dark Blue',0.08,0.2,0.34);
#10629=FILL_AREA_STYLE_COLOUR('',#10628);
#10630=FILL_AREA_STYLE('',(#10629));
#10631=SURFACE_STYLE_FILL_AREA(#10630);
#10632=SURFACE_SIDE_STYLE('',(#10631));
#10633=SURFACE_STYLE_USAGE(.BOTH.,#10632);
#10634=PRESENTATION_STYLE_ASSIGNMENT((#10633));
ENDSEC;
END-ISO-10303-21;
